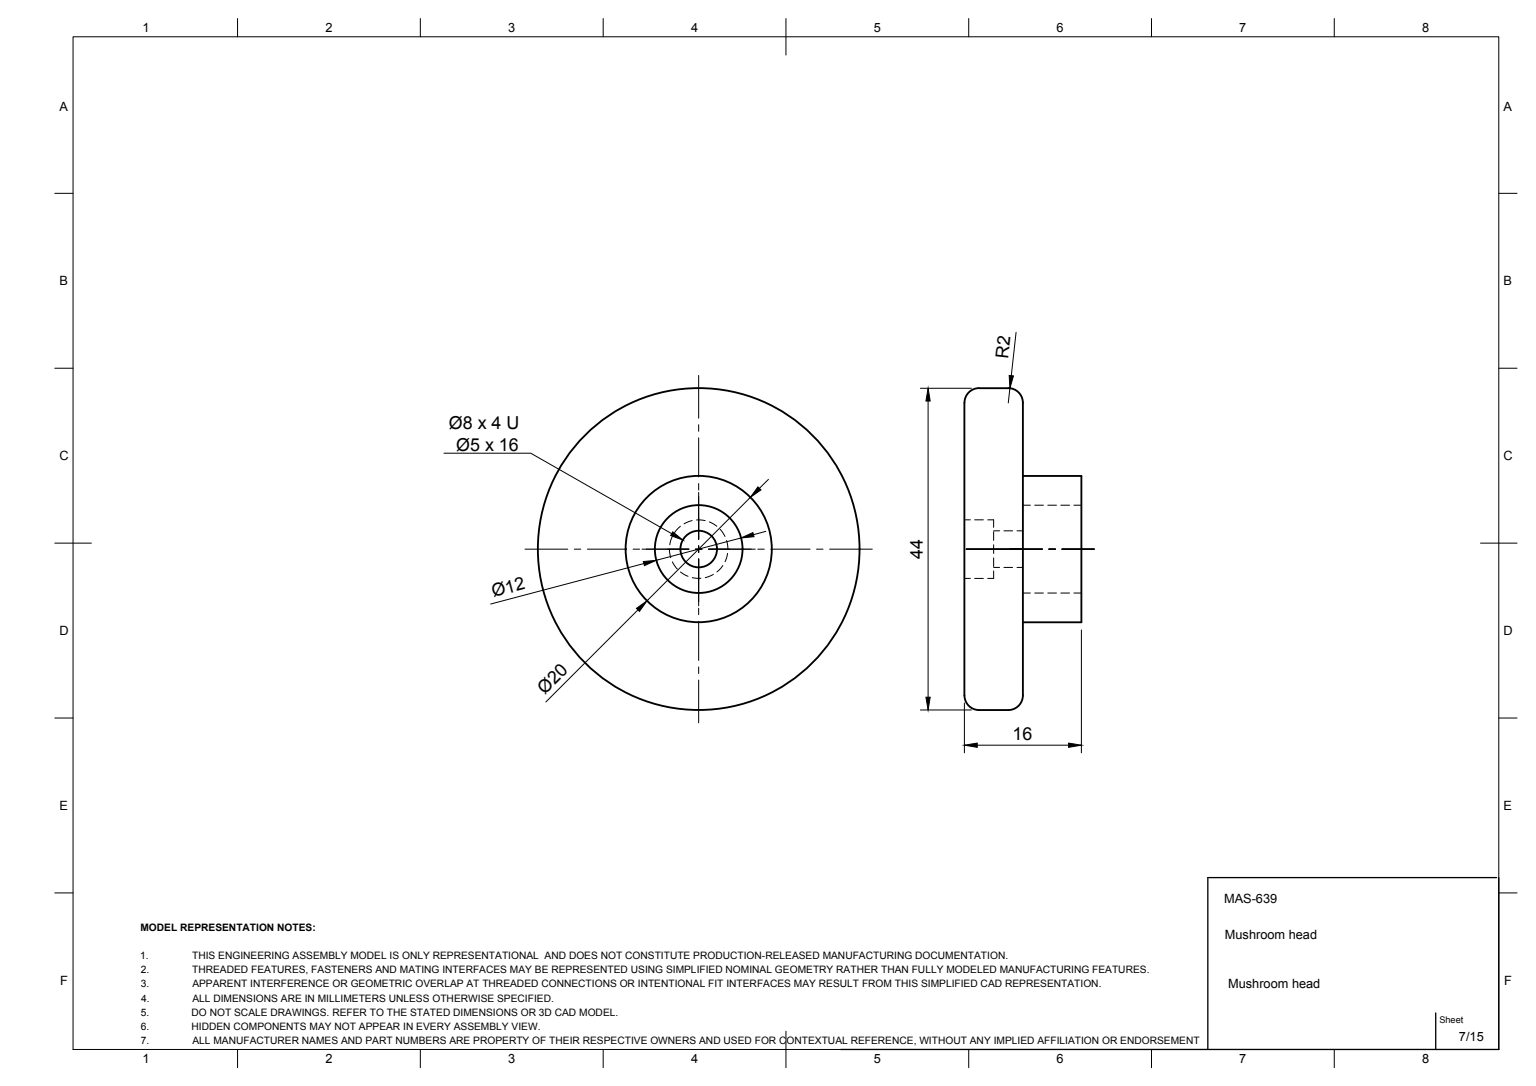
ISO-10303-21;
HEADER;
/* Generated by software containing ST-Developer
 * from STEP Tools, Inc. (www.steptools.com) 
 */

FILE_DESCRIPTION(
/* description */ ('Independent maintained push-to-latch/pull-to-reset mushroom-operator 
CAD. Two opposed spring-loaded ball detents in turned circular seats b
ias both travel stops; direct normally-closed bridge opens6mm when pre
ssed. Rounded palm/pull rim, captured head screw, removable detent clo
sures, native Coil spring families, insulated shared terminals and ord
inary machining features. Manual geometric states and ideal same-mater
ial spring-energy direction only; no electrical/safety certification, 
force/contact dynamics, wear, load or life rating. Requested blue/gray
 visual palette, not safety identification. External wiring/anchors an
d application engineering omitted.'),
/* implementation_level */ '2;1');

FILE_NAME(
/* name */ 'Mushroom head.step',
/* time_stamp */ '2026-11-08T17:54:26-08:00',
/* author */ (''),
/* organization */ (''),
/* preprocessor_version */ 'ST-DEVELOPER v20.2',
/* originating_system */ 'Autodesk Translation Framework v15.17.0.0',
/* authorisation */ '');

FILE_SCHEMA (('AUTOMOTIVE_DESIGN { 1 0 10303 214 3 1 1 }'));
ENDSEC;

DATA;
#10=MECHANICAL_DESIGN_GEOMETRIC_PRESENTATION_REPRESENTATION('',(#194),#43980);
#154=TOROIDAL_SURFACE('',#11852,2.,0.2);
#155=TOROIDAL_SURFACE('',#11860,2.,0.2);
#160=SHAPE_REPRESENTATION_RELATIONSHIP('SRR','None',#44060,#177);
#177=ADVANCED_BREP_SHAPE_REPRESENTATION('',(#211),#43967);
#194=STYLED_ITEM('',(#44150),#211);
#211=MANIFOLD_SOLID_BREP('Body1',#11235);
#306=FACE_BOUND('',#1470,.T.);
#307=FACE_BOUND('',#1473,.T.);
#308=FACE_BOUND('',#1475,.T.);
#309=FACE_BOUND('',#1478,.T.);
#310=FACE_BOUND('',#1483,.T.);
#400=PLANE('',#11858);
#401=PLANE('',#11863);
#402=PLANE('',#11865);
#403=PLANE('',#11869);
#404=PLANE('',#11877);
#797=FACE_OUTER_BOUND('',#1467,.T.);
#798=FACE_OUTER_BOUND('',#1468,.T.);
#799=FACE_OUTER_BOUND('',#1469,.T.);
#800=FACE_OUTER_BOUND('',#1471,.T.);
#801=FACE_OUTER_BOUND('',#1472,.T.);
#802=FACE_OUTER_BOUND('',#1474,.T.);
#803=FACE_OUTER_BOUND('',#1476,.T.);
#804=FACE_OUTER_BOUND('',#1477,.T.);
#805=FACE_OUTER_BOUND('',#1479,.T.);
#806=FACE_OUTER_BOUND('',#1480,.T.);
#807=FACE_OUTER_BOUND('',#1481,.T.);
#808=FACE_OUTER_BOUND('',#1482,.T.);
#1467=EDGE_LOOP('',(#8571,#8572,#8573,#8574));
#1468=EDGE_LOOP('',(#8575,#8576,#8577,#8578));
#1469=EDGE_LOOP('',(#8579));
#1470=EDGE_LOOP('',(#8580));
#1471=EDGE_LOOP('',(#8581,#8582,#8583,#8584));
#1472=EDGE_LOOP('',(#8585));
#1473=EDGE_LOOP('',(#8586));
#1474=EDGE_LOOP('',(#8587));
#1475=EDGE_LOOP('',(#8588));
#1476=EDGE_LOOP('',(#8589,#8590,#8591,#8592));
#1477=EDGE_LOOP('',(#8593));
#1478=EDGE_LOOP('',(#8594));
#1479=EDGE_LOOP('',(#8595,#8596,#8597,#8598));
#1480=EDGE_LOOP('',(#8599,#8600,#8601,#8602));
#1481=EDGE_LOOP('',(#8603,#8604,#8605,#8606));
#1482=EDGE_LOOP('',(#8607));
#1483=EDGE_LOOP('',(#8608));
#1916=CIRCLE('',#11853,2.);
#1917=CIRCLE('',#11854,0.2);
#1918=CIRCLE('',#11855,2.2);
#1919=CIRCLE('',#11857,2.2);
#1920=CIRCLE('',#11859,0.4);
#1921=CIRCLE('',#11861,0.2);
#1922=CIRCLE('',#11862,2.);
#1923=CIRCLE('',#11864,1.);
#1924=CIRCLE('',#11866,0.4);
#1925=CIRCLE('',#11867,0.25);
#1926=CIRCLE('',#11870,0.6);
#1927=CIRCLE('',#11871,0.25);
#1928=CIRCLE('',#11874,0.6);
#1929=CIRCLE('',#11876,1.);
#3141=LINE('',#29323,#3773);
#3142=LINE('',#29341,#3774);
#3143=LINE('',#29348,#3775);
#3144=LINE('',#29351,#3776);
#3145=LINE('',#29355,#3777);
#3773=VECTOR('',#13420,2.2);
#3774=VECTOR('',#13445,0.4);
#3775=VECTOR('',#13454,0.25);
#3776=VECTOR('',#13457,0.6);
#3777=VECTOR('',#13462,1.);
#4662=VERTEX_POINT('',#29316);
#4663=VERTEX_POINT('',#29318);
#4664=VERTEX_POINT('',#29322);
#4665=VERTEX_POINT('',#29326);
#4666=VERTEX_POINT('',#29329);
#4667=VERTEX_POINT('',#29333);
#4668=VERTEX_POINT('',#29336);
#4669=VERTEX_POINT('',#29338);
#4670=VERTEX_POINT('',#29343);
#4671=VERTEX_POINT('',#29345);
#4672=VERTEX_POINT('',#29350);
#4673=VERTEX_POINT('',#29354);
#6055=EDGE_CURVE('',#4662,#4662,#1916,.T.);
#6056=EDGE_CURVE('',#4662,#4663,#1917,.T.);
#6057=EDGE_CURVE('',#4663,#4663,#1918,.T.);
#6058=EDGE_CURVE('',#4663,#4664,#3141,.T.);
#6059=EDGE_CURVE('',#4664,#4664,#1919,.T.);
#6060=EDGE_CURVE('',#4665,#4665,#1920,.T.);
#6061=EDGE_CURVE('',#4664,#4666,#1921,.T.);
#6062=EDGE_CURVE('',#4666,#4666,#1922,.T.);
#6063=EDGE_CURVE('',#4667,#4667,#1923,.T.);
#6064=EDGE_CURVE('',#4668,#4668,#1924,.T.);
#6065=EDGE_CURVE('',#4669,#4669,#1925,.T.);
#6066=EDGE_CURVE('',#4665,#4668,#3142,.T.);
#6067=EDGE_CURVE('',#4670,#4670,#1926,.T.);
#6068=EDGE_CURVE('',#4671,#4671,#1927,.T.);
#6069=EDGE_CURVE('',#4669,#4671,#3143,.T.);
#6070=EDGE_CURVE('',#4670,#4672,#3144,.T.);
#6071=EDGE_CURVE('',#4672,#4672,#1928,.T.);
#6072=EDGE_CURVE('',#4667,#4673,#3145,.T.);
#6073=EDGE_CURVE('',#4673,#4673,#1929,.T.);
#8571=ORIENTED_EDGE('',*,*,#6055,.T.);
#8572=ORIENTED_EDGE('',*,*,#6056,.T.);
#8573=ORIENTED_EDGE('',*,*,#6057,.T.);
#8574=ORIENTED_EDGE('',*,*,#6056,.F.);
#8575=ORIENTED_EDGE('',*,*,#6057,.F.);
#8576=ORIENTED_EDGE('',*,*,#6058,.T.);
#8577=ORIENTED_EDGE('',*,*,#6059,.F.);
#8578=ORIENTED_EDGE('',*,*,#6058,.F.);
#8579=ORIENTED_EDGE('',*,*,#6055,.F.);
#8580=ORIENTED_EDGE('',*,*,#6060,.T.);
#8581=ORIENTED_EDGE('',*,*,#6059,.T.);
#8582=ORIENTED_EDGE('',*,*,#6061,.T.);
#8583=ORIENTED_EDGE('',*,*,#6062,.T.);
#8584=ORIENTED_EDGE('',*,*,#6061,.F.);
#8585=ORIENTED_EDGE('',*,*,#6062,.F.);
#8586=ORIENTED_EDGE('',*,*,#6063,.T.);
#8587=ORIENTED_EDGE('',*,*,#6064,.F.);
#8588=ORIENTED_EDGE('',*,*,#6065,.F.);
#8589=ORIENTED_EDGE('',*,*,#6060,.F.);
#8590=ORIENTED_EDGE('',*,*,#6066,.T.);
#8591=ORIENTED_EDGE('',*,*,#6064,.T.);
#8592=ORIENTED_EDGE('',*,*,#6066,.F.);
#8593=ORIENTED_EDGE('',*,*,#6067,.T.);
#8594=ORIENTED_EDGE('',*,*,#6068,.F.);
#8595=ORIENTED_EDGE('',*,*,#6065,.T.);
#8596=ORIENTED_EDGE('',*,*,#6069,.T.);
#8597=ORIENTED_EDGE('',*,*,#6068,.T.);
#8598=ORIENTED_EDGE('',*,*,#6069,.F.);
#8599=ORIENTED_EDGE('',*,*,#6067,.F.);
#8600=ORIENTED_EDGE('',*,*,#6070,.T.);
#8601=ORIENTED_EDGE('',*,*,#6071,.T.);
#8602=ORIENTED_EDGE('',*,*,#6070,.F.);
#8603=ORIENTED_EDGE('',*,*,#6063,.F.);
#8604=ORIENTED_EDGE('',*,*,#6072,.T.);
#8605=ORIENTED_EDGE('',*,*,#6073,.T.);
#8606=ORIENTED_EDGE('',*,*,#6072,.F.);
#8607=ORIENTED_EDGE('',*,*,#6073,.F.);
#8608=ORIENTED_EDGE('',*,*,#6071,.F.);
#10407=CYLINDRICAL_SURFACE('',#11856,2.2);
#10408=CYLINDRICAL_SURFACE('',#11868,0.4);
#10409=CYLINDRICAL_SURFACE('',#11872,0.25);
#10410=CYLINDRICAL_SURFACE('',#11873,0.6);
#10411=CYLINDRICAL_SURFACE('',#11875,1.);
#10922=ADVANCED_FACE('',(#797),#154,.T.);
#10923=ADVANCED_FACE('',(#798),#10407,.T.);
#10924=ADVANCED_FACE('',(#799,#306),#400,.T.);
#10925=ADVANCED_FACE('',(#800),#155,.T.);
#10926=ADVANCED_FACE('',(#801,#307),#401,.F.);
#10927=ADVANCED_FACE('',(#802,#308),#402,.F.);
#10928=ADVANCED_FACE('',(#803),#10408,.F.);
#10929=ADVANCED_FACE('',(#804,#309),#403,.F.);
#10930=ADVANCED_FACE('',(#805),#10409,.F.);
#10931=ADVANCED_FACE('',(#806),#10410,.F.);
#10932=ADVANCED_FACE('',(#807),#10411,.T.);
#10933=ADVANCED_FACE('',(#808,#310),#404,.F.);
#11235=CLOSED_SHELL('',(#10922,#10923,#10924,#10925,#10926,#10927,#10928,
#10929,#10930,#10931,#10932,#10933));
#11851=AXIS2_PLACEMENT_3D('',#29314,#13408,#13409);
#11852=AXIS2_PLACEMENT_3D('',#29315,#13410,#13411);
#11853=AXIS2_PLACEMENT_3D('',#29317,#13412,#13413);
#11854=AXIS2_PLACEMENT_3D('',#29319,#13414,#13415);
#11855=AXIS2_PLACEMENT_3D('',#29320,#13416,#13417);
#11856=AXIS2_PLACEMENT_3D('',#29321,#13418,#13419);
#11857=AXIS2_PLACEMENT_3D('',#29324,#13421,#13422);
#11858=AXIS2_PLACEMENT_3D('',#29325,#13423,#13424);
#11859=AXIS2_PLACEMENT_3D('',#29327,#13425,#13426);
#11860=AXIS2_PLACEMENT_3D('',#29328,#13427,#13428);
#11861=AXIS2_PLACEMENT_3D('',#29330,#13429,#13430);
#11862=AXIS2_PLACEMENT_3D('',#29331,#13431,#13432);
#11863=AXIS2_PLACEMENT_3D('',#29332,#13433,#13434);
#11864=AXIS2_PLACEMENT_3D('',#29334,#13435,#13436);
#11865=AXIS2_PLACEMENT_3D('',#29335,#13437,#13438);
#11866=AXIS2_PLACEMENT_3D('',#29337,#13439,#13440);
#11867=AXIS2_PLACEMENT_3D('',#29339,#13441,#13442);
#11868=AXIS2_PLACEMENT_3D('',#29340,#13443,#13444);
#11869=AXIS2_PLACEMENT_3D('',#29342,#13446,#13447);
#11870=AXIS2_PLACEMENT_3D('',#29344,#13448,#13449);
#11871=AXIS2_PLACEMENT_3D('',#29346,#13450,#13451);
#11872=AXIS2_PLACEMENT_3D('',#29347,#13452,#13453);
#11873=AXIS2_PLACEMENT_3D('',#29349,#13455,#13456);
#11874=AXIS2_PLACEMENT_3D('',#29352,#13458,#13459);
#11875=AXIS2_PLACEMENT_3D('',#29353,#13460,#13461);
#11876=AXIS2_PLACEMENT_3D('',#29356,#13463,#13464);
#11877=AXIS2_PLACEMENT_3D('',#29357,#13465,#13466);
#13408=DIRECTION('axis',(0.,0.,1.));
#13409=DIRECTION('refdir',(1.,0.,0.));
#13410=DIRECTION('center_axis',(0.,0.,1.));
#13411=DIRECTION('ref_axis',(1.,0.,0.));
#13412=DIRECTION('center_axis',(0.,0.,-1.));
#13413=DIRECTION('ref_axis',(1.,0.,0.));
#13414=DIRECTION('center_axis',(1.22464679914735E-16,-1.,0.));
#13415=DIRECTION('ref_axis',(-1.,-1.22464679914735E-16,0.));
#13416=DIRECTION('center_axis',(0.,0.,1.));
#13417=DIRECTION('ref_axis',(1.,0.,0.));
#13418=DIRECTION('center_axis',(0.,0.,1.));
#13419=DIRECTION('ref_axis',(1.,0.,0.));
#13420=DIRECTION('',(0.,0.,-1.));
#13421=DIRECTION('center_axis',(0.,0.,-1.));
#13422=DIRECTION('ref_axis',(1.,0.,0.));
#13423=DIRECTION('center_axis',(0.,0.,1.));
#13424=DIRECTION('ref_axis',(1.,0.,0.));
#13425=DIRECTION('center_axis',(0.,0.,-1.));
#13426=DIRECTION('ref_axis',(1.,0.,0.));
#13427=DIRECTION('center_axis',(0.,0.,1.));
#13428=DIRECTION('ref_axis',(1.,0.,0.));
#13429=DIRECTION('center_axis',(1.22464679914735E-16,-1.,0.));
#13430=DIRECTION('ref_axis',(-1.,-1.22464679914735E-16,0.));
#13431=DIRECTION('center_axis',(0.,0.,1.));
#13432=DIRECTION('ref_axis',(1.,0.,0.));
#13433=DIRECTION('center_axis',(0.,0.,1.));
#13434=DIRECTION('ref_axis',(1.,0.,0.));
#13435=DIRECTION('center_axis',(0.,0.,1.));
#13436=DIRECTION('ref_axis',(1.,0.,0.));
#13437=DIRECTION('center_axis',(0.,0.,-1.));
#13438=DIRECTION('ref_axis',(1.,0.,0.));
#13439=DIRECTION('center_axis',(0.,0.,-1.));
#13440=DIRECTION('ref_axis',(1.,0.,0.));
#13441=DIRECTION('center_axis',(0.,0.,1.));
#13442=DIRECTION('ref_axis',(1.,0.,0.));
#13443=DIRECTION('center_axis',(0.,0.,-1.));
#13444=DIRECTION('ref_axis',(1.,0.,0.));
#13445=DIRECTION('',(0.,0.,-1.));
#13446=DIRECTION('center_axis',(0.,0.,1.));
#13447=DIRECTION('ref_axis',(1.,0.,0.));
#13448=DIRECTION('center_axis',(0.,0.,-1.));
#13449=DIRECTION('ref_axis',(1.,0.,0.));
#13450=DIRECTION('center_axis',(0.,0.,-1.));
#13451=DIRECTION('ref_axis',(1.,0.,0.));
#13452=DIRECTION('center_axis',(0.,0.,1.));
#13453=DIRECTION('ref_axis',(1.,0.,0.));
#13454=DIRECTION('',(0.,0.,-1.));
#13455=DIRECTION('center_axis',(0.,0.,1.));
#13456=DIRECTION('ref_axis',(1.,0.,0.));
#13457=DIRECTION('',(0.,0.,-1.));
#13458=DIRECTION('center_axis',(0.,0.,-1.));
#13459=DIRECTION('ref_axis',(1.,0.,0.));
#13460=DIRECTION('center_axis',(0.,0.,1.));
#13461=DIRECTION('ref_axis',(1.,0.,0.));
#13462=DIRECTION('',(0.,0.,-1.));
#13463=DIRECTION('center_axis',(0.,0.,1.));
#13464=DIRECTION('ref_axis',(1.,0.,0.));
#13465=DIRECTION('center_axis',(0.,0.,1.));
#13466=DIRECTION('ref_axis',(1.,0.,0.));
#29314=CARTESIAN_POINT('',(0.,0.,0.));
#29315=CARTESIAN_POINT('Origin',(0.,0.,9.2));
#29316=CARTESIAN_POINT('',(-2.,2.44929359829471E-16,9.4));
#29317=CARTESIAN_POINT('Origin',(0.,0.,9.4));
#29318=CARTESIAN_POINT('',(-2.2,-2.69422295812418E-16,9.2));
#29319=CARTESIAN_POINT('Origin',(-2.,-2.44929359829471E-16,9.2));
#29320=CARTESIAN_POINT('Origin',(0.,0.,9.2));
#29321=CARTESIAN_POINT('Origin',(0.,0.,8.6));
#29322=CARTESIAN_POINT('',(-2.2,2.69422295812418E-16,8.8));
#29323=CARTESIAN_POINT('',(-2.2,-2.69422295812418E-16,8.6));
#29324=CARTESIAN_POINT('Origin',(0.,0.,8.8));
#29325=CARTESIAN_POINT('Origin',(0.,0.,9.4));
#29326=CARTESIAN_POINT('',(-0.4,4.89858719658941E-17,9.4));
#29327=CARTESIAN_POINT('Origin',(0.,0.,9.4));
#29328=CARTESIAN_POINT('Origin',(0.,0.,8.8));
#29329=CARTESIAN_POINT('',(-2.,-2.44929359829471E-16,8.6));
#29330=CARTESIAN_POINT('Origin',(-2.,-2.44929359829471E-16,8.8));
#29331=CARTESIAN_POINT('Origin',(0.,0.,8.6));
#29332=CARTESIAN_POINT('Origin',(0.,0.,8.6));
#29333=CARTESIAN_POINT('',(-1.,-1.22464679914735E-16,8.6));
#29334=CARTESIAN_POINT('Origin',(0.,0.,8.6));
#29335=CARTESIAN_POINT('Origin',(0.,0.,9.));
#29336=CARTESIAN_POINT('',(-0.4,4.89858719658941E-17,9.));
#29337=CARTESIAN_POINT('Origin',(0.,0.,9.));
#29338=CARTESIAN_POINT('',(-0.25,3.06161699786838E-17,9.));
#29339=CARTESIAN_POINT('Origin',(0.,0.,9.));
#29340=CARTESIAN_POINT('Origin',(0.,0.,9.2));
#29341=CARTESIAN_POINT('',(-0.4,4.89858719658941E-17,9.2));
#29342=CARTESIAN_POINT('Origin',(0.,0.,8.6));
#29343=CARTESIAN_POINT('',(-0.6,-7.34788079488412E-17,8.6));
#29344=CARTESIAN_POINT('Origin',(0.,0.,8.6));
#29345=CARTESIAN_POINT('',(-0.25,-3.06161699786838E-17,8.6));
#29346=CARTESIAN_POINT('Origin',(0.,0.,8.6));
#29347=CARTESIAN_POINT('Origin',(0.,0.,8.6));
#29348=CARTESIAN_POINT('',(-0.25,-3.06161699786838E-17,8.6));
#29349=CARTESIAN_POINT('Origin',(0.,0.,7.8));
#29350=CARTESIAN_POINT('',(-0.6,-7.34788079488412E-17,7.8));
#29351=CARTESIAN_POINT('',(-0.6,-7.34788079488412E-17,7.8));
#29352=CARTESIAN_POINT('Origin',(0.,0.,7.8));
#29353=CARTESIAN_POINT('Origin',(0.,0.,7.8));
#29354=CARTESIAN_POINT('',(-1.,-1.22464679914735E-16,7.8));
#29355=CARTESIAN_POINT('',(-1.,-1.22464679914735E-16,7.8));
#29356=CARTESIAN_POINT('Origin',(0.,0.,7.8));
#29357=CARTESIAN_POINT('Origin',(0.,0.,7.8));
#43948=UNCERTAINTY_MEASURE_WITH_UNIT(LENGTH_MEASURE(0.001),#43981,
'DISTANCE_ACCURACY_VALUE',
'Maximum model space distance between geometric entities at asserted c
onnectivities');
#43961=UNCERTAINTY_MEASURE_WITH_UNIT(LENGTH_MEASURE(0.001),#43981,
'DISTANCE_ACCURACY_VALUE',
'Maximum model space distance between geometric entities at asserted c
onnectivities');
#43967=(
GEOMETRIC_REPRESENTATION_CONTEXT(3)
GLOBAL_UNCERTAINTY_ASSIGNED_CONTEXT((#43948))
GLOBAL_UNIT_ASSIGNED_CONTEXT((#43981,#43983,#43984))
REPRESENTATION_CONTEXT('','3D')
);
#43980=(
GEOMETRIC_REPRESENTATION_CONTEXT(3)
GLOBAL_UNCERTAINTY_ASSIGNED_CONTEXT((#43961))
GLOBAL_UNIT_ASSIGNED_CONTEXT((#43981,#43983,#43984))
REPRESENTATION_CONTEXT('','3D')
);
#43981=(
LENGTH_UNIT()
NAMED_UNIT(*)
SI_UNIT(.CENTI.,.METRE.)
);
#43983=(
NAMED_UNIT(*)
PLANE_ANGLE_UNIT()
SI_UNIT($,.RADIAN.)
);
#43984=(
NAMED_UNIT(*)
SI_UNIT($,.STERADIAN.)
SOLID_ANGLE_UNIT()
);
#43990=SHAPE_DEFINITION_REPRESENTATION(#44008,#44060);
#44008=PRODUCT_DEFINITION_SHAPE('',$,#44079);
#44060=SHAPE_REPRESENTATION('',(#11851),#43967);
#44073=PRODUCT_DEFINITION_CONTEXT('part definition',#44129,'design');
#44079=PRODUCT_DEFINITION('Mushroom head','Mushroom head',#44097,#44073);
#44097=PRODUCT_DEFINITION_FORMATION('',$,#44136);
#44129=APPLICATION_CONTEXT(
'Core Data for Automotive Mechanical Design Process');
#44130=PRODUCT_CONTEXT('part definition',#44129,'mechanical');
#44136=PRODUCT('Mushroom head','Mushroom head',$,(#44130));
#44150=PRESENTATION_STYLE_ASSIGNMENT((#44162));
#44162=SURFACE_STYLE_USAGE(.BOTH.,#44174);
#44174=SURFACE_SIDE_STYLE('',(#44186));
#44186=SURFACE_STYLE_FILL_AREA(#44198);
#44198=FILL_AREA_STYLE('Dark blue',(#44210));
#44210=FILL_AREA_STYLE_COLOUR('Dark blue',#44222);
#44222=COLOUR_RGB('Dark blue',0.0901960784313725,0.270588235294118,0.513725490196078);
ENDSEC;
END-ISO-10303-21;
